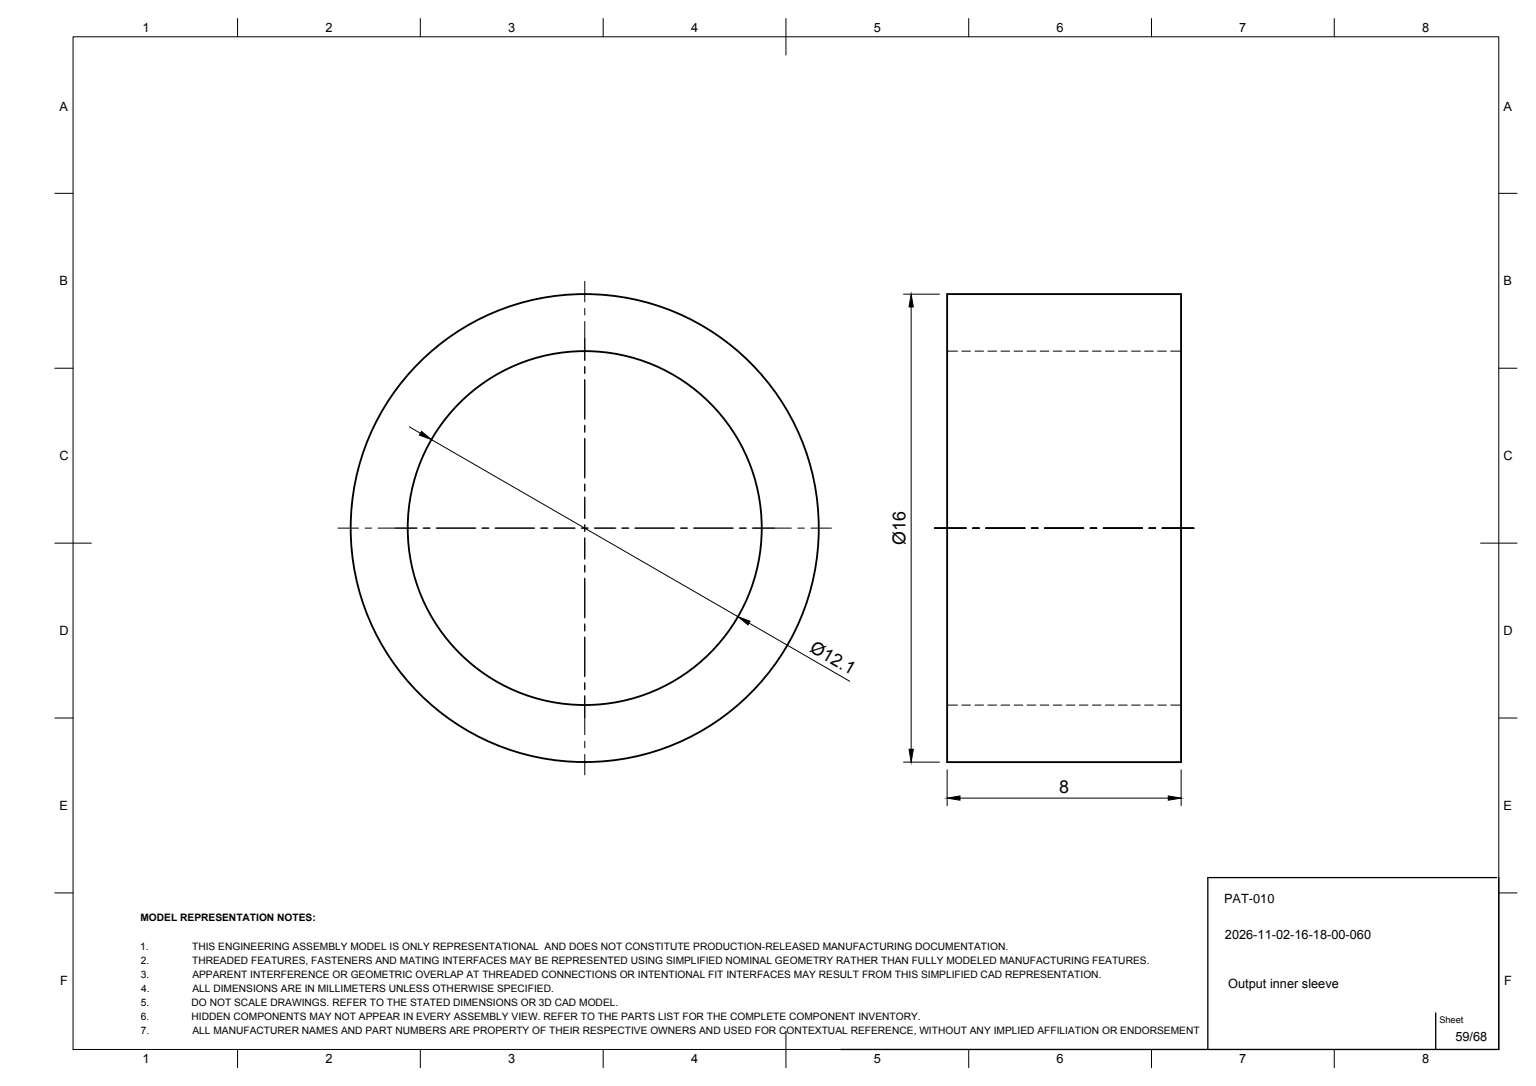
ISO-10303-21;
HEADER;
/* Generated by software containing ST-Developer
 * from STEP Tools, Inc. (www.steptools.com) 
 */

FILE_DESCRIPTION(
/* description */ ('Belt conveyor head drive unit'),
/* implementation_level */ '2;1');

FILE_NAME(
/* name */ 'Output inner sleeve.step',
/* time_stamp */ '2026-10-28T03:26:19-07:00',
/* author */ (''),
/* organization */ (''),
/* preprocessor_version */ 'ST-DEVELOPER v20.2',
/* originating_system */ 'Autodesk Translation Framework v15.17.0.0',
/* authorisation */ '');

FILE_SCHEMA (('AUTOMOTIVE_DESIGN { 1 0 10303 214 3 1 1 }'));
ENDSEC;

DATA;
#10=MECHANICAL_DESIGN_GEOMETRIC_PRESENTATION_REPRESENTATION('',(#918),#27069);
#764=SHAPE_REPRESENTATION_RELATIONSHIP('SRR','None',#27413,#833);
#833=ADVANCED_BREP_SHAPE_REPRESENTATION('',(#999),#27055);
#918=STYLED_ITEM('',(#27790),#999);
#999=MANIFOLD_SOLID_BREP('Body1',#13787);
#1238=FACE_BOUND('',#3286,.T.);
#1239=FACE_BOUND('',#3288,.T.);
#1578=PLANE('',#15906);
#1579=PLANE('',#15907);
#2257=FACE_OUTER_BOUND('',#3283,.T.);
#2258=FACE_OUTER_BOUND('',#3284,.T.);
#2259=FACE_OUTER_BOUND('',#3285,.T.);
#2260=FACE_OUTER_BOUND('',#3287,.T.);
#3283=EDGE_LOOP('',(#11658,#11659,#11660,#11661));
#3284=EDGE_LOOP('',(#11662,#11663,#11664,#11665));
#3285=EDGE_LOOP('',(#11666));
#3286=EDGE_LOOP('',(#11667));
#3287=EDGE_LOOP('',(#11668));
#3288=EDGE_LOOP('',(#11669));
#4123=LINE('',#25369,#4915);
#4124=LINE('',#25375,#4916);
#4915=VECTOR('',#19739,0.605);
#4916=VECTOR('',#19746,0.8);
#5721=CIRCLE('',#15901,0.605);
#5722=CIRCLE('',#15902,0.605);
#5723=CIRCLE('',#15904,0.8);
#5724=CIRCLE('',#15905,0.8);
#6877=VERTEX_POINT('',#25366);
#6878=VERTEX_POINT('',#25368);
#6879=VERTEX_POINT('',#25372);
#6880=VERTEX_POINT('',#25374);
#8521=EDGE_CURVE('',#6877,#6877,#5721,.T.);
#8522=EDGE_CURVE('',#6877,#6878,#4123,.T.);
#8523=EDGE_CURVE('',#6878,#6878,#5722,.T.);
#8524=EDGE_CURVE('',#6879,#6879,#5723,.T.);
#8525=EDGE_CURVE('',#6879,#6880,#4124,.T.);
#8526=EDGE_CURVE('',#6880,#6880,#5724,.T.);
#11658=ORIENTED_EDGE('',*,*,#8521,.F.);
#11659=ORIENTED_EDGE('',*,*,#8522,.T.);
#11660=ORIENTED_EDGE('',*,*,#8523,.T.);
#11661=ORIENTED_EDGE('',*,*,#8522,.F.);
#11662=ORIENTED_EDGE('',*,*,#8524,.F.);
#11663=ORIENTED_EDGE('',*,*,#8525,.T.);
#11664=ORIENTED_EDGE('',*,*,#8526,.T.);
#11665=ORIENTED_EDGE('',*,*,#8525,.F.);
#11666=ORIENTED_EDGE('',*,*,#8524,.T.);
#11667=ORIENTED_EDGE('',*,*,#8521,.T.);
#11668=ORIENTED_EDGE('',*,*,#8526,.F.);
#11669=ORIENTED_EDGE('',*,*,#8523,.F.);
#12797=CYLINDRICAL_SURFACE('',#15900,0.605);
#12798=CYLINDRICAL_SURFACE('',#15903,0.8);
#13536=ADVANCED_FACE('',(#2257),#12797,.F.);
#13537=ADVANCED_FACE('',(#2258),#12798,.T.);
#13538=ADVANCED_FACE('',(#2259,#1238),#1578,.T.);
#13539=ADVANCED_FACE('',(#2260,#1239),#1579,.F.);
#13787=CLOSED_SHELL('',(#13536,#13537,#13538,#13539));
#15899=AXIS2_PLACEMENT_3D('',#25364,#19733,#19734);
#15900=AXIS2_PLACEMENT_3D('',#25365,#19735,#19736);
#15901=AXIS2_PLACEMENT_3D('',#25367,#19737,#19738);
#15902=AXIS2_PLACEMENT_3D('',#25370,#19740,#19741);
#15903=AXIS2_PLACEMENT_3D('',#25371,#19742,#19743);
#15904=AXIS2_PLACEMENT_3D('',#25373,#19744,#19745);
#15905=AXIS2_PLACEMENT_3D('',#25376,#19747,#19748);
#15906=AXIS2_PLACEMENT_3D('',#25377,#19749,#19750);
#15907=AXIS2_PLACEMENT_3D('',#25378,#19751,#19752);
#19733=DIRECTION('axis',(0.,0.,1.));
#19734=DIRECTION('refdir',(1.,0.,0.));
#19735=DIRECTION('center_axis',(0.,1.,0.));
#19736=DIRECTION('ref_axis',(1.,0.,0.));
#19737=DIRECTION('center_axis',(0.,-1.,0.));
#19738=DIRECTION('ref_axis',(1.,0.,0.));
#19739=DIRECTION('',(0.,-1.,0.));
#19740=DIRECTION('center_axis',(0.,-1.,0.));
#19741=DIRECTION('ref_axis',(1.,0.,0.));
#19742=DIRECTION('center_axis',(0.,1.,0.));
#19743=DIRECTION('ref_axis',(1.,0.,0.));
#19744=DIRECTION('center_axis',(0.,1.,0.));
#19745=DIRECTION('ref_axis',(1.,0.,0.));
#19746=DIRECTION('',(0.,-1.,0.));
#19747=DIRECTION('center_axis',(0.,1.,0.));
#19748=DIRECTION('ref_axis',(1.,0.,0.));
#19749=DIRECTION('center_axis',(0.,1.,0.));
#19750=DIRECTION('ref_axis',(1.,0.,0.));
#19751=DIRECTION('center_axis',(0.,1.,0.));
#19752=DIRECTION('ref_axis',(1.,0.,0.));
#25364=CARTESIAN_POINT('',(0.,0.,0.));
#25365=CARTESIAN_POINT('Origin',(6.97091003018116,-0.4,7.));
#25366=CARTESIAN_POINT('',(6.36591003018116,0.4,7.));
#25367=CARTESIAN_POINT('Origin',(6.97091003018116,0.4,7.));
#25368=CARTESIAN_POINT('',(6.36591003018116,-0.4,7.));
#25369=CARTESIAN_POINT('',(6.36591003018116,-0.4,7.));
#25370=CARTESIAN_POINT('Origin',(6.97091003018116,-0.4,7.));
#25371=CARTESIAN_POINT('Origin',(6.97091003018116,-0.4,7.));
#25372=CARTESIAN_POINT('',(6.17091003018116,0.4,7.));
#25373=CARTESIAN_POINT('Origin',(6.97091003018116,0.4,7.));
#25374=CARTESIAN_POINT('',(6.17091003018116,-0.4,7.));
#25375=CARTESIAN_POINT('',(6.17091003018116,-0.4,7.));
#25376=CARTESIAN_POINT('Origin',(6.97091003018116,-0.4,7.));
#25377=CARTESIAN_POINT('Origin',(6.97091003018116,0.4,7.));
#25378=CARTESIAN_POINT('Origin',(6.97091003018116,-0.4,7.));
#26978=UNCERTAINTY_MEASURE_WITH_UNIT(LENGTH_MEASURE(0.001),#27070,
'DISTANCE_ACCURACY_VALUE',
'Maximum model space distance between geometric entities at asserted c
onnectivities');
#26992=UNCERTAINTY_MEASURE_WITH_UNIT(LENGTH_MEASURE(0.001),#27070,
'DISTANCE_ACCURACY_VALUE',
'Maximum model space distance between geometric entities at asserted c
onnectivities');
#27055=(
GEOMETRIC_REPRESENTATION_CONTEXT(3)
GLOBAL_UNCERTAINTY_ASSIGNED_CONTEXT((#26978))
GLOBAL_UNIT_ASSIGNED_CONTEXT((#27070,#27072,#27073))
REPRESENTATION_CONTEXT('','3D')
);
#27069=(
GEOMETRIC_REPRESENTATION_CONTEXT(3)
GLOBAL_UNCERTAINTY_ASSIGNED_CONTEXT((#26992))
GLOBAL_UNIT_ASSIGNED_CONTEXT((#27070,#27072,#27073))
REPRESENTATION_CONTEXT('','3D')
);
#27070=(
LENGTH_UNIT()
NAMED_UNIT(*)
SI_UNIT(.CENTI.,.METRE.)
);
#27072=(
NAMED_UNIT(*)
PLANE_ANGLE_UNIT()
SI_UNIT($,.RADIAN.)
);
#27073=(
NAMED_UNIT(*)
SI_UNIT($,.STERADIAN.)
SOLID_ANGLE_UNIT()
);
#27136=SHAPE_DEFINITION_REPRESENTATION(#27224,#27413);
#27224=PRODUCT_DEFINITION_SHAPE('',$,#27490);
#27413=SHAPE_REPRESENTATION('',(#15899),#27055);
#27427=PRODUCT_DEFINITION_CONTEXT('part definition',#27657,'design');
#27490=PRODUCT_DEFINITION('Output inner sleeve','Output inner sleeve',#27566,
#27427);
#27566=PRODUCT_DEFINITION_FORMATION('',$,#27721);
#27657=APPLICATION_CONTEXT(
'Core Data for Automotive Mechanical Design Process');
#27658=PRODUCT_CONTEXT('part definition',#27657,'mechanical');
#27721=PRODUCT('Output inner sleeve','Output inner sleeve',
'Output inner sleeve',(#27658));
#27784=COLOUR_RGB('Sky Blue',0.24,0.69,0.87);
#27785=FILL_AREA_STYLE_COLOUR('',#27784);
#27786=FILL_AREA_STYLE('',(#27785));
#27787=SURFACE_STYLE_FILL_AREA(#27786);
#27788=SURFACE_SIDE_STYLE('',(#27787));
#27789=SURFACE_STYLE_USAGE(.BOTH.,#27788);
#27790=PRESENTATION_STYLE_ASSIGNMENT((#27789));
ENDSEC;
END-ISO-10303-21;
